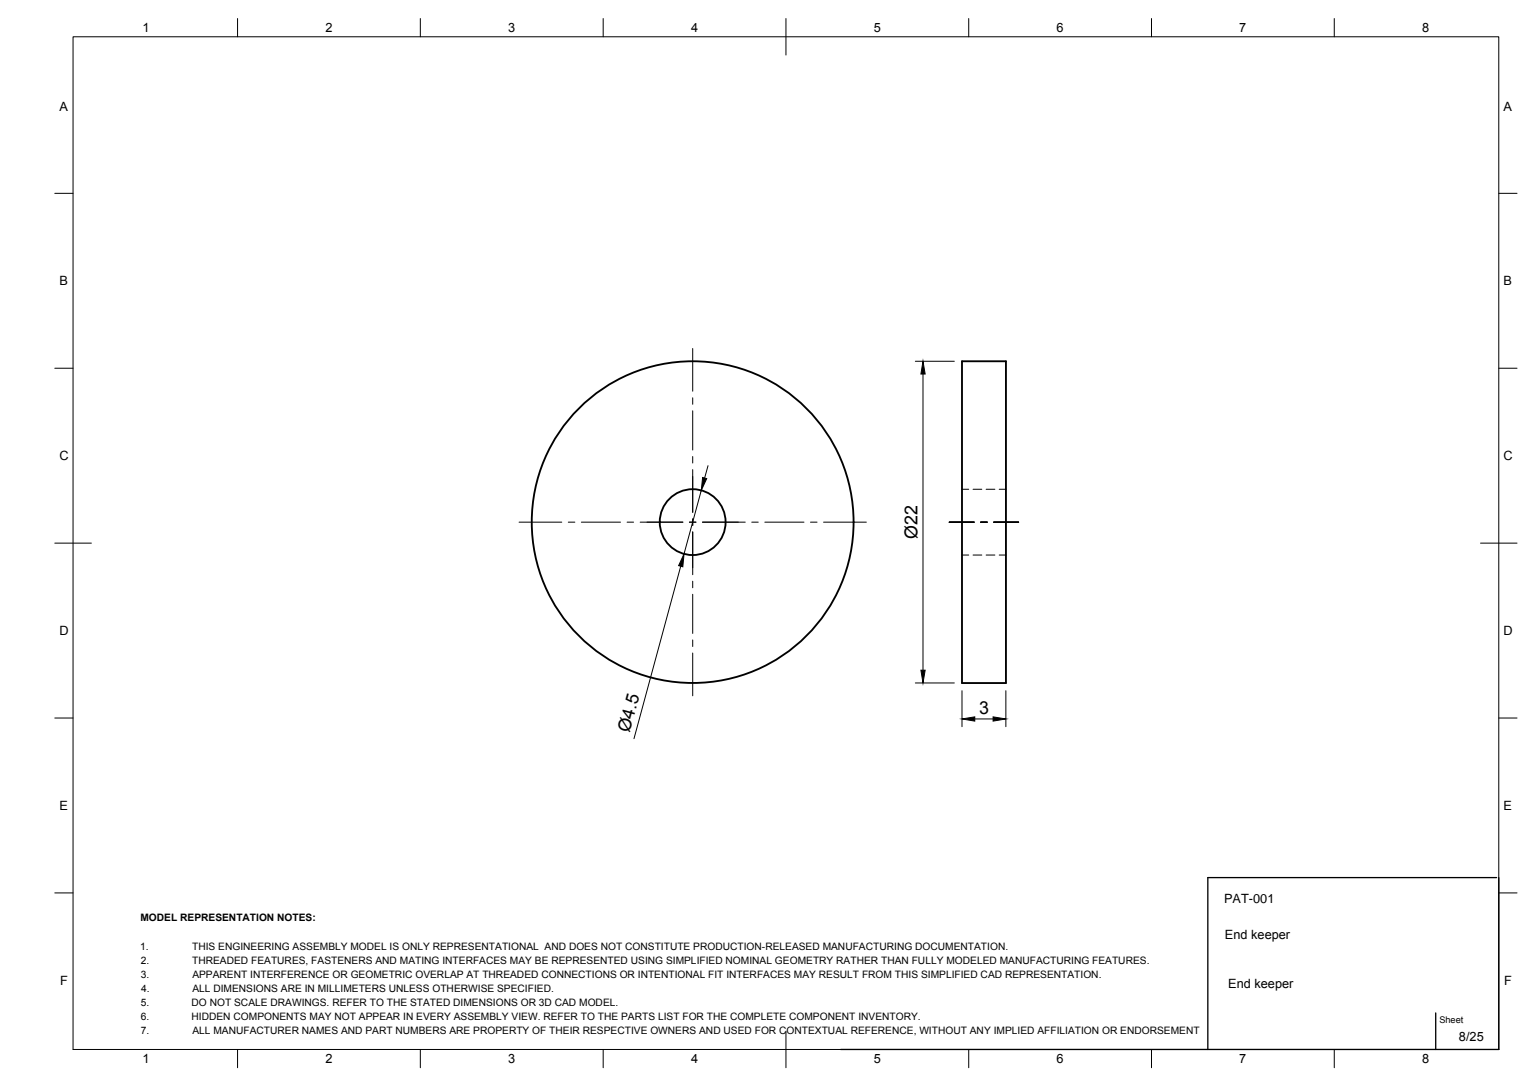
ISO-10303-21;
HEADER;
/* Generated by software containing ST-Developer
 * from STEP Tools, Inc. (www.steptools.com) 
 */

FILE_DESCRIPTION(
/* description */ ('PAT-001'),
/* implementation_level */ '2;1');

FILE_NAME(
/* name */ 'End keeper.step',
/* time_stamp */ '2026-10-29T17:07:15-07:00',
/* author */ (''),
/* organization */ (''),
/* preprocessor_version */ 'ST-DEVELOPER v20.2',
/* originating_system */ 'Autodesk Translation Framework v15.17.0.0',
/* authorisation */ '');

FILE_SCHEMA (('AUTOMOTIVE_DESIGN { 1 0 10303 214 3 1 1 }'));
ENDSEC;

DATA;
#10=MECHANICAL_DESIGN_GEOMETRIC_PRESENTATION_REPRESENTATION('',(#376),#9622);
#326=SHAPE_REPRESENTATION_RELATIONSHIP('SRR','None',#9749,#351);
#351=ADVANCED_BREP_SHAPE_REPRESENTATION('',(#409),#9598);
#376=STYLED_ITEM('',(#9976),#409);
#409=MANIFOLD_SOLID_BREP('Body1',#5201);
#445=FACE_BOUND('',#1041,.T.);
#446=FACE_BOUND('',#1043,.T.);
#538=PLANE('',#5558);
#539=PLANE('',#5559);
#734=FACE_OUTER_BOUND('',#1038,.T.);
#735=FACE_OUTER_BOUND('',#1039,.T.);
#736=FACE_OUTER_BOUND('',#1040,.T.);
#737=FACE_OUTER_BOUND('',#1042,.T.);
#1038=EDGE_LOOP('',(#3571,#3572,#3573,#3574));
#1039=EDGE_LOOP('',(#3575,#3576,#3577,#3578));
#1040=EDGE_LOOP('',(#3579));
#1041=EDGE_LOOP('',(#3580));
#1042=EDGE_LOOP('',(#3581));
#1043=EDGE_LOOP('',(#3582));
#1407=LINE('',#7782,#1812);
#1408=LINE('',#7788,#1813);
#1812=VECTOR('',#6206,0.225);
#1813=VECTOR('',#6213,1.1);
#2226=CIRCLE('',#5553,0.225);
#2227=CIRCLE('',#5554,0.225);
#2228=CIRCLE('',#5556,1.1);
#2229=CIRCLE('',#5557,1.1);
#2438=VERTEX_POINT('',#7779);
#2439=VERTEX_POINT('',#7781);
#2440=VERTEX_POINT('',#7785);
#2441=VERTEX_POINT('',#7787);
#2889=EDGE_CURVE('',#2438,#2438,#2226,.T.);
#2890=EDGE_CURVE('',#2438,#2439,#1407,.T.);
#2891=EDGE_CURVE('',#2439,#2439,#2227,.T.);
#2892=EDGE_CURVE('',#2440,#2440,#2228,.T.);
#2893=EDGE_CURVE('',#2440,#2441,#1408,.T.);
#2894=EDGE_CURVE('',#2441,#2441,#2229,.T.);
#3571=ORIENTED_EDGE('',*,*,#2889,.F.);
#3572=ORIENTED_EDGE('',*,*,#2890,.T.);
#3573=ORIENTED_EDGE('',*,*,#2891,.T.);
#3574=ORIENTED_EDGE('',*,*,#2890,.F.);
#3575=ORIENTED_EDGE('',*,*,#2892,.F.);
#3576=ORIENTED_EDGE('',*,*,#2893,.T.);
#3577=ORIENTED_EDGE('',*,*,#2894,.T.);
#3578=ORIENTED_EDGE('',*,*,#2893,.F.);
#3579=ORIENTED_EDGE('',*,*,#2892,.T.);
#3580=ORIENTED_EDGE('',*,*,#2889,.T.);
#3581=ORIENTED_EDGE('',*,*,#2894,.F.);
#3582=ORIENTED_EDGE('',*,*,#2891,.F.);
#4836=CYLINDRICAL_SURFACE('',#5552,0.225);
#4837=CYLINDRICAL_SURFACE('',#5555,1.1);
#4921=ADVANCED_FACE('',(#734),#4836,.F.);
#4922=ADVANCED_FACE('',(#735),#4837,.T.);
#4923=ADVANCED_FACE('',(#736,#445),#538,.T.);
#4924=ADVANCED_FACE('',(#737,#446),#539,.F.);
#5201=CLOSED_SHELL('',(#4921,#4922,#4923,#4924));
#5551=AXIS2_PLACEMENT_3D('',#7777,#6200,#6201);
#5552=AXIS2_PLACEMENT_3D('',#7778,#6202,#6203);
#5553=AXIS2_PLACEMENT_3D('',#7780,#6204,#6205);
#5554=AXIS2_PLACEMENT_3D('',#7783,#6207,#6208);
#5555=AXIS2_PLACEMENT_3D('',#7784,#6209,#6210);
#5556=AXIS2_PLACEMENT_3D('',#7786,#6211,#6212);
#5557=AXIS2_PLACEMENT_3D('',#7789,#6214,#6215);
#5558=AXIS2_PLACEMENT_3D('',#7790,#6216,#6217);
#5559=AXIS2_PLACEMENT_3D('',#7791,#6218,#6219);
#6200=DIRECTION('axis',(0.,0.,1.));
#6201=DIRECTION('refdir',(1.,0.,0.));
#6202=DIRECTION('center_axis',(0.,1.,0.));
#6203=DIRECTION('ref_axis',(1.,0.,0.));
#6204=DIRECTION('center_axis',(0.,-1.,0.));
#6205=DIRECTION('ref_axis',(1.,0.,0.));
#6206=DIRECTION('',(0.,-1.,0.));
#6207=DIRECTION('center_axis',(0.,-1.,0.));
#6208=DIRECTION('ref_axis',(1.,0.,0.));
#6209=DIRECTION('center_axis',(0.,1.,0.));
#6210=DIRECTION('ref_axis',(1.,0.,0.));
#6211=DIRECTION('center_axis',(0.,1.,0.));
#6212=DIRECTION('ref_axis',(1.,0.,0.));
#6213=DIRECTION('',(0.,-1.,0.));
#6214=DIRECTION('center_axis',(0.,1.,0.));
#6215=DIRECTION('ref_axis',(1.,0.,0.));
#6216=DIRECTION('center_axis',(0.,1.,0.));
#6217=DIRECTION('ref_axis',(1.,0.,0.));
#6218=DIRECTION('center_axis',(0.,1.,0.));
#6219=DIRECTION('ref_axis',(1.,0.,0.));
#7777=CARTESIAN_POINT('',(0.,0.,0.));
#7778=CARTESIAN_POINT('Origin',(0.,-2.8,4.5));
#7779=CARTESIAN_POINT('',(-0.225,-2.5,4.5));
#7780=CARTESIAN_POINT('Origin',(0.,-2.5,4.5));
#7781=CARTESIAN_POINT('',(-0.225,-2.8,4.5));
#7782=CARTESIAN_POINT('',(-0.225,-2.8,4.5));
#7783=CARTESIAN_POINT('Origin',(0.,-2.8,4.5));
#7784=CARTESIAN_POINT('Origin',(0.,-2.8,4.5));
#7785=CARTESIAN_POINT('',(-1.1,-2.5,4.5));
#7786=CARTESIAN_POINT('Origin',(0.,-2.5,4.5));
#7787=CARTESIAN_POINT('',(-1.1,-2.8,4.5));
#7788=CARTESIAN_POINT('',(-1.1,-2.8,4.5));
#7789=CARTESIAN_POINT('Origin',(0.,-2.8,4.5));
#7790=CARTESIAN_POINT('Origin',(0.,-2.5,4.5));
#7791=CARTESIAN_POINT('Origin',(0.,-2.8,4.5));
#9568=UNCERTAINTY_MEASURE_WITH_UNIT(LENGTH_MEASURE(0.001),#9623,
'DISTANCE_ACCURACY_VALUE',
'Maximum model space distance between geometric entities at asserted c
onnectivities');
#9592=UNCERTAINTY_MEASURE_WITH_UNIT(LENGTH_MEASURE(0.001),#9623,
'DISTANCE_ACCURACY_VALUE',
'Maximum model space distance between geometric entities at asserted c
onnectivities');
#9598=(
GEOMETRIC_REPRESENTATION_CONTEXT(3)
GLOBAL_UNCERTAINTY_ASSIGNED_CONTEXT((#9568))
GLOBAL_UNIT_ASSIGNED_CONTEXT((#9623,#9625,#9626))
REPRESENTATION_CONTEXT('','3D')
);
#9622=(
GEOMETRIC_REPRESENTATION_CONTEXT(3)
GLOBAL_UNCERTAINTY_ASSIGNED_CONTEXT((#9592))
GLOBAL_UNIT_ASSIGNED_CONTEXT((#9623,#9625,#9626))
REPRESENTATION_CONTEXT('','3D')
);
#9623=(
LENGTH_UNIT()
NAMED_UNIT(*)
SI_UNIT(.CENTI.,.METRE.)
);
#9625=(
NAMED_UNIT(*)
PLANE_ANGLE_UNIT()
SI_UNIT($,.RADIAN.)
);
#9626=(
NAMED_UNIT(*)
SI_UNIT($,.STERADIAN.)
SOLID_ANGLE_UNIT()
);
#9632=SHAPE_DEFINITION_REPRESENTATION(#9661,#9749);
#9661=PRODUCT_DEFINITION_SHAPE('',$,#9779);
#9749=SHAPE_REPRESENTATION('',(#5551),#9598);
#9773=PRODUCT_DEFINITION_CONTEXT('part definition',#9862,'design');
#9779=PRODUCT_DEFINITION('End keeper','End keeper',#9808,#9773);
#9808=PRODUCT_DEFINITION_FORMATION('',$,#9869);
#9862=APPLICATION_CONTEXT(
'Core Data for Automotive Mechanical Design Process');
#9863=PRODUCT_CONTEXT('part definition',#9862,'mechanical');
#9869=PRODUCT('End keeper','End keeper','End keeper',(#9863));
#9970=COLOUR_RGB('Off White',0.89,0.88,0.83);
#9971=FILL_AREA_STYLE_COLOUR('',#9970);
#9972=FILL_AREA_STYLE('',(#9971));
#9973=SURFACE_STYLE_FILL_AREA(#9972);
#9974=SURFACE_SIDE_STYLE('',(#9973));
#9975=SURFACE_STYLE_USAGE(.BOTH.,#9974);
#9976=PRESENTATION_STYLE_ASSIGNMENT((#9975));
ENDSEC;
END-ISO-10303-21;
